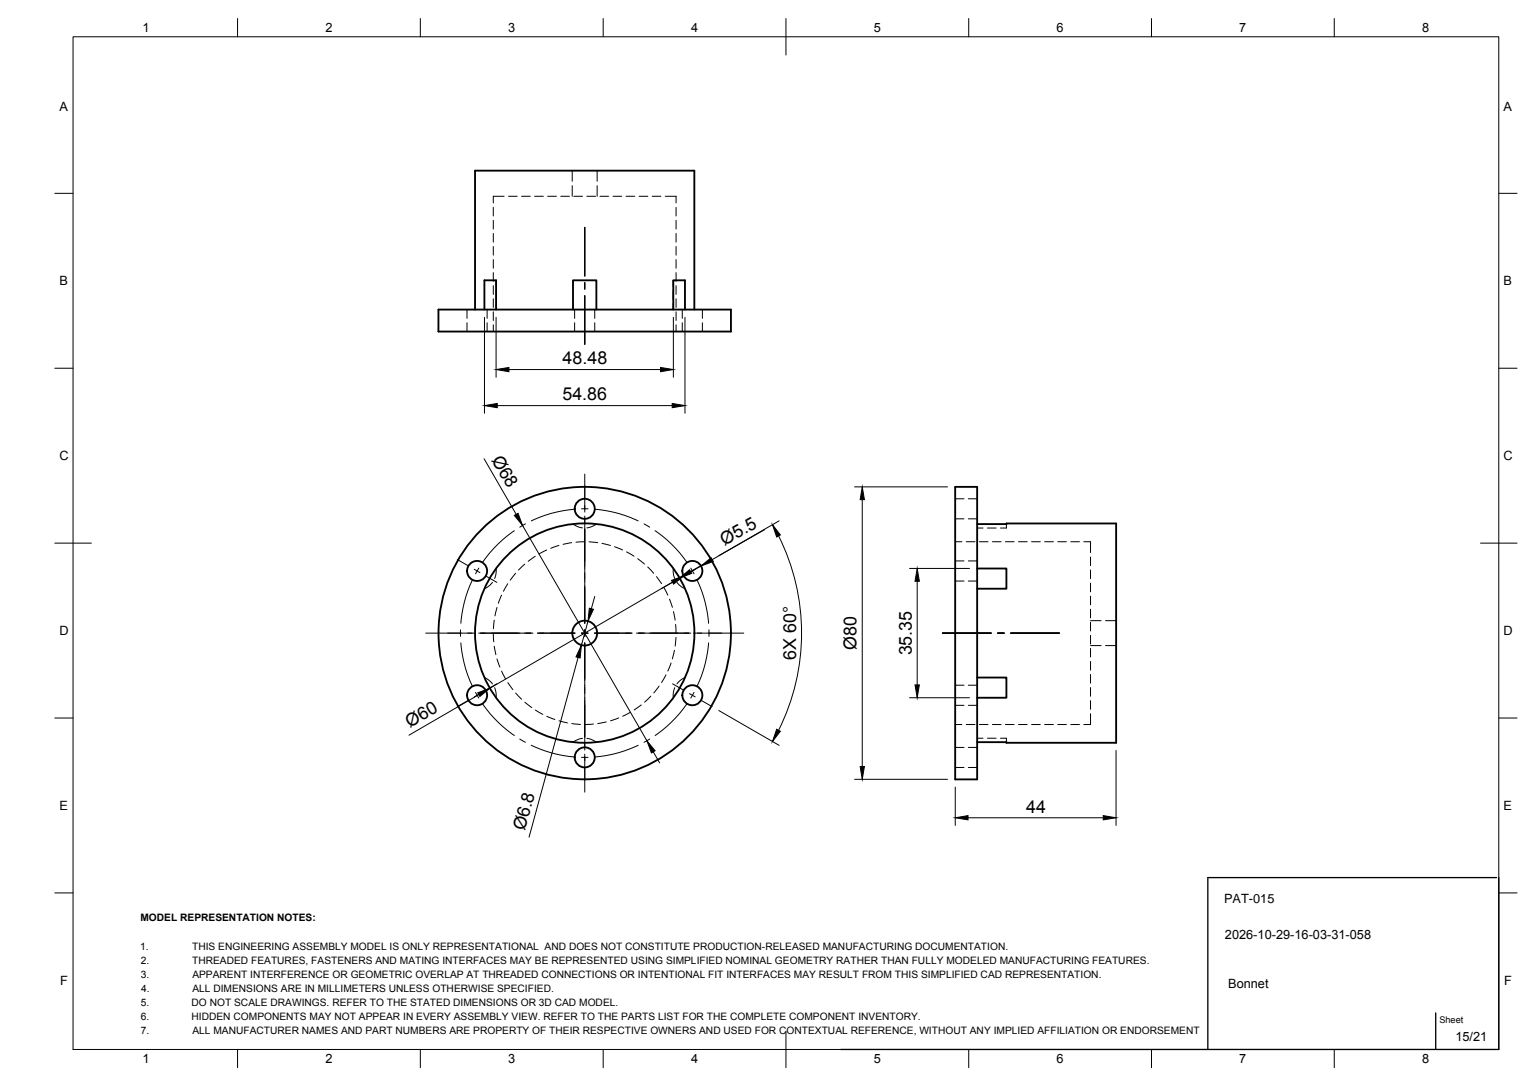
ISO-10303-21;
HEADER;
/* Generated by software containing ST-Developer
 * from STEP Tools, Inc. (www.steptools.com) 
 */

FILE_DESCRIPTION(
/* description */ ('PAT-015'),
/* implementation_level */ '2;1');

FILE_NAME(
/* name */ 'Bonnet.step',
/* time_stamp */ '2026-10-29T16:03:43-07:00',
/* author */ (''),
/* organization */ (''),
/* preprocessor_version */ 'ST-DEVELOPER v20.2',
/* originating_system */ 'Autodesk Translation Framework v15.17.0.0',
/* authorisation */ '');

FILE_SCHEMA (('AUTOMOTIVE_DESIGN { 1 0 10303 214 3 1 1 }'));
ENDSEC;

DATA;
#10=MECHANICAL_DESIGN_GEOMETRIC_PRESENTATION_REPRESENTATION('',(#243),#10266);
#195=SHAPE_REPRESENTATION_RELATIONSHIP('SRR','None',#10366,#218);
#218=ADVANCED_BREP_SHAPE_REPRESENTATION('',(#268),#10254);
#243=STYLED_ITEM('',(#10540),#268);
#268=MANIFOLD_SOLID_BREP('Body1',#4702);
#390=FACE_BOUND('',#1144,.T.);
#391=FACE_BOUND('',#1146,.T.);
#392=FACE_BOUND('',#1149,.T.);
#393=FACE_BOUND('',#1150,.T.);
#394=FACE_BOUND('',#1151,.T.);
#395=FACE_BOUND('',#1152,.T.);
#396=FACE_BOUND('',#1153,.T.);
#397=FACE_BOUND('',#1154,.T.);
#398=FACE_BOUND('',#1155,.T.);
#399=FACE_BOUND('',#1157,.T.);
#400=FACE_BOUND('',#1158,.T.);
#401=FACE_BOUND('',#1159,.T.);
#402=FACE_BOUND('',#1160,.T.);
#403=FACE_BOUND('',#1161,.T.);
#404=FACE_BOUND('',#1162,.T.);
#405=FACE_BOUND('',#1163,.T.);
#503=PLANE('',#5307);
#504=PLANE('',#5315);
#505=PLANE('',#5317);
#506=PLANE('',#5322);
#507=PLANE('',#5327);
#508=PLANE('',#5335);
#509=PLANE('',#5370);
#510=PLANE('',#5371);
#511=PLANE('',#5375);
#512=PLANE('',#5376);
#741=FACE_OUTER_BOUND('',#1122,.T.);
#742=FACE_OUTER_BOUND('',#1123,.T.);
#743=FACE_OUTER_BOUND('',#1124,.T.);
#744=FACE_OUTER_BOUND('',#1125,.T.);
#745=FACE_OUTER_BOUND('',#1126,.T.);
#746=FACE_OUTER_BOUND('',#1127,.T.);
#747=FACE_OUTER_BOUND('',#1128,.T.);
#748=FACE_OUTER_BOUND('',#1129,.T.);
#749=FACE_OUTER_BOUND('',#1130,.T.);
#750=FACE_OUTER_BOUND('',#1131,.T.);
#751=FACE_OUTER_BOUND('',#1132,.T.);
#752=FACE_OUTER_BOUND('',#1133,.T.);
#753=FACE_OUTER_BOUND('',#1134,.T.);
#754=FACE_OUTER_BOUND('',#1135,.T.);
#755=FACE_OUTER_BOUND('',#1136,.T.);
#756=FACE_OUTER_BOUND('',#1137,.T.);
#757=FACE_OUTER_BOUND('',#1138,.T.);
#758=FACE_OUTER_BOUND('',#1139,.T.);
#759=FACE_OUTER_BOUND('',#1140,.T.);
#760=FACE_OUTER_BOUND('',#1141,.T.);
#761=FACE_OUTER_BOUND('',#1142,.T.);
#762=FACE_OUTER_BOUND('',#1143,.T.);
#763=FACE_OUTER_BOUND('',#1145,.T.);
#764=FACE_OUTER_BOUND('',#1147,.T.);
#765=FACE_OUTER_BOUND('',#1148,.T.);
#766=FACE_OUTER_BOUND('',#1156,.T.);
#1122=EDGE_LOOP('',(#3831,#3832));
#1123=EDGE_LOOP('',(#3833,#3834,#3835,#3836));
#1124=EDGE_LOOP('',(#3837,#3838,#3839,#3840));
#1125=EDGE_LOOP('',(#3841,#3842));
#1126=EDGE_LOOP('',(#3843,#3844));
#1127=EDGE_LOOP('',(#3845,#3846,#3847,#3848));
#1128=EDGE_LOOP('',(#3849,#3850));
#1129=EDGE_LOOP('',(#3851,#3852,#3853,#3854));
#1130=EDGE_LOOP('',(#3855,#3856));
#1131=EDGE_LOOP('',(#3857,#3858,#3859,#3860));
#1132=EDGE_LOOP('',(#3861,#3862,#3863,#3864));
#1133=EDGE_LOOP('',(#3865,#3866));
#1134=EDGE_LOOP('',(#3867,#3868,#3869,#3870,#3871,#3872,#3873,#3874,#3875,
#3876,#3877,#3878,#3879,#3880,#3881,#3882,#3883,#3884,#3885,#3886,#3887,
#3888,#3889,#3890,#3891,#3892,#3893,#3894));
#1135=EDGE_LOOP('',(#3895,#3896,#3897,#3898));
#1136=EDGE_LOOP('',(#3899,#3900,#3901,#3902));
#1137=EDGE_LOOP('',(#3903,#3904,#3905,#3906));
#1138=EDGE_LOOP('',(#3907,#3908,#3909,#3910));
#1139=EDGE_LOOP('',(#3911,#3912,#3913,#3914));
#1140=EDGE_LOOP('',(#3915,#3916,#3917,#3918));
#1141=EDGE_LOOP('',(#3919,#3920,#3921,#3922));
#1142=EDGE_LOOP('',(#3923,#3924,#3925,#3926));
#1143=EDGE_LOOP('',(#3927));
#1144=EDGE_LOOP('',(#3928));
#1145=EDGE_LOOP('',(#3929));
#1146=EDGE_LOOP('',(#3930));
#1147=EDGE_LOOP('',(#3931,#3932,#3933,#3934));
#1148=EDGE_LOOP('',(#3935));
#1149=EDGE_LOOP('',(#3936));
#1150=EDGE_LOOP('',(#3937));
#1151=EDGE_LOOP('',(#3938));
#1152=EDGE_LOOP('',(#3939));
#1153=EDGE_LOOP('',(#3940));
#1154=EDGE_LOOP('',(#3941));
#1155=EDGE_LOOP('',(#3942,#3943,#3944,#3945,#3946,#3947,#3948,#3949,#3950,
#3951,#3952,#3953,#3954));
#1156=EDGE_LOOP('',(#3955));
#1157=EDGE_LOOP('',(#3956));
#1158=EDGE_LOOP('',(#3957));
#1159=EDGE_LOOP('',(#3958));
#1160=EDGE_LOOP('',(#3959));
#1161=EDGE_LOOP('',(#3960));
#1162=EDGE_LOOP('',(#3961));
#1163=EDGE_LOOP('',(#3962));
#1480=LINE('',#8832,#1760);
#1481=LINE('',#8835,#1761);
#1482=LINE('',#8839,#1762);
#1483=LINE('',#8843,#1763);
#1484=LINE('',#8854,#1764);
#1485=LINE('',#8857,#1765);
#1486=LINE('',#8865,#1766);
#1487=LINE('',#8868,#1767);
#1488=LINE('',#8876,#1768);
#1489=LINE('',#8879,#1769);
#1490=LINE('',#8883,#1770);
#1491=LINE('',#8887,#1771);
#1492=LINE('',#8895,#1772);
#1493=LINE('',#8907,#1773);
#1494=LINE('',#8913,#1774);
#1495=LINE('',#8919,#1775);
#1496=LINE('',#8925,#1776);
#1497=LINE('',#8931,#1777);
#1498=LINE('',#8937,#1778);
#1499=LINE('',#8943,#1779);
#1500=LINE('',#8949,#1780);
#1501=LINE('',#8957,#1781);
#1760=VECTOR('',#6395,1.);
#1761=VECTOR('',#6398,1.);
#1762=VECTOR('',#6401,1.);
#1763=VECTOR('',#6404,1.);
#1764=VECTOR('',#6419,1.);
#1765=VECTOR('',#6422,1.);
#1766=VECTOR('',#6431,1.);
#1767=VECTOR('',#6434,1.);
#1768=VECTOR('',#6443,1.);
#1769=VECTOR('',#6446,1.);
#1770=VECTOR('',#6449,1.);
#1771=VECTOR('',#6452,1.);
#1772=VECTOR('',#6463,3.);
#1773=VECTOR('',#6482,0.275);
#1774=VECTOR('',#6489,0.275);
#1775=VECTOR('',#6496,0.275);
#1776=VECTOR('',#6503,0.275);
#1777=VECTOR('',#6510,0.275);
#1778=VECTOR('',#6517,0.275);
#1779=VECTOR('',#6524,0.34);
#1780=VECTOR('',#6531,2.5);
#1781=VECTOR('',#6542,4.);
#2023=CIRCLE('',#5308,3.);
#2024=CIRCLE('',#5309,0.525);
#2025=CIRCLE('',#5311,0.525);
#2026=CIRCLE('',#5313,0.525);
#2027=CIRCLE('',#5314,0.525);
#2028=CIRCLE('',#5316,3.);
#2029=CIRCLE('',#5318,3.);
#2030=CIRCLE('',#5319,0.525);
#2031=CIRCLE('',#5321,0.525);
#2032=CIRCLE('',#5323,3.);
#2033=CIRCLE('',#5324,0.525);
#2034=CIRCLE('',#5326,0.525);
#2035=CIRCLE('',#5328,3.);
#2036=CIRCLE('',#5329,0.525);
#2037=CIRCLE('',#5331,0.525);
#2038=CIRCLE('',#5333,0.525);
#2039=CIRCLE('',#5334,0.525);
#2040=CIRCLE('',#5336,3.);
#2041=CIRCLE('',#5338,3.);
#2042=CIRCLE('',#5339,3.);
#2043=CIRCLE('',#5340,3.);
#2044=CIRCLE('',#5341,3.);
#2045=CIRCLE('',#5342,3.);
#2046=CIRCLE('',#5343,3.);
#2047=CIRCLE('',#5344,3.);
#2048=CIRCLE('',#5345,3.);
#2049=CIRCLE('',#5347,0.275);
#2050=CIRCLE('',#5348,0.275);
#2051=CIRCLE('',#5350,0.275);
#2052=CIRCLE('',#5351,0.275);
#2053=CIRCLE('',#5353,0.275);
#2054=CIRCLE('',#5354,0.275);
#2055=CIRCLE('',#5356,0.275);
#2056=CIRCLE('',#5357,0.275);
#2057=CIRCLE('',#5359,0.275);
#2058=CIRCLE('',#5360,0.275);
#2059=CIRCLE('',#5362,0.275);
#2060=CIRCLE('',#5363,0.275);
#2061=CIRCLE('',#5365,0.34);
#2062=CIRCLE('',#5366,0.34);
#2063=CIRCLE('',#5368,2.5);
#2064=CIRCLE('',#5369,2.5);
#2065=CIRCLE('',#5373,4.);
#2066=CIRCLE('',#5374,4.);
#2357=VERTEX_POINT('',#8826);
#2358=VERTEX_POINT('',#8827);
#2359=VERTEX_POINT('',#8831);
#2360=VERTEX_POINT('',#8833);
#2361=VERTEX_POINT('',#8837);
#2362=VERTEX_POINT('',#8838);
#2363=VERTEX_POINT('',#8840);
#2364=VERTEX_POINT('',#8842);
#2365=VERTEX_POINT('',#8848);
#2366=VERTEX_POINT('',#8849);
#2367=VERTEX_POINT('',#8853);
#2368=VERTEX_POINT('',#8855);
#2369=VERTEX_POINT('',#8859);
#2370=VERTEX_POINT('',#8860);
#2371=VERTEX_POINT('',#8864);
#2372=VERTEX_POINT('',#8866);
#2373=VERTEX_POINT('',#8870);
#2374=VERTEX_POINT('',#8871);
#2375=VERTEX_POINT('',#8875);
#2376=VERTEX_POINT('',#8877);
#2377=VERTEX_POINT('',#8881);
#2378=VERTEX_POINT('',#8882);
#2379=VERTEX_POINT('',#8884);
#2380=VERTEX_POINT('',#8886);
#2381=VERTEX_POINT('',#8892);
#2382=VERTEX_POINT('',#8894);
#2383=VERTEX_POINT('',#8904);
#2384=VERTEX_POINT('',#8906);
#2385=VERTEX_POINT('',#8910);
#2386=VERTEX_POINT('',#8912);
#2387=VERTEX_POINT('',#8916);
#2388=VERTEX_POINT('',#8918);
#2389=VERTEX_POINT('',#8922);
#2390=VERTEX_POINT('',#8924);
#2391=VERTEX_POINT('',#8928);
#2392=VERTEX_POINT('',#8930);
#2393=VERTEX_POINT('',#8934);
#2394=VERTEX_POINT('',#8936);
#2395=VERTEX_POINT('',#8940);
#2396=VERTEX_POINT('',#8942);
#2397=VERTEX_POINT('',#8946);
#2398=VERTEX_POINT('',#8948);
#2399=VERTEX_POINT('',#8954);
#2400=VERTEX_POINT('',#8956);
#2871=EDGE_CURVE('',#2357,#2358,#2023,.T.);
#2872=EDGE_CURVE('',#2358,#2357,#2024,.T.);
#2873=EDGE_CURVE('',#2359,#2357,#1480,.T.);
#2874=EDGE_CURVE('',#2360,#2359,#2025,.T.);
#2875=EDGE_CURVE('',#2358,#2360,#1481,.T.);
#2876=EDGE_CURVE('',#2361,#2362,#1482,.T.);
#2877=EDGE_CURVE('',#2361,#2363,#2026,.T.);
#2878=EDGE_CURVE('',#2364,#2363,#1483,.T.);
#2879=EDGE_CURVE('',#2362,#2364,#2027,.T.);
#2880=EDGE_CURVE('',#2363,#2361,#2028,.T.);
#2881=EDGE_CURVE('',#2365,#2366,#2029,.T.);
#2882=EDGE_CURVE('',#2366,#2365,#2030,.T.);
#2883=EDGE_CURVE('',#2367,#2365,#1484,.T.);
#2884=EDGE_CURVE('',#2368,#2367,#2031,.T.);
#2885=EDGE_CURVE('',#2366,#2368,#1485,.T.);
#2886=EDGE_CURVE('',#2369,#2370,#2032,.T.);
#2887=EDGE_CURVE('',#2370,#2369,#2033,.T.);
#2888=EDGE_CURVE('',#2371,#2369,#1486,.T.);
#2889=EDGE_CURVE('',#2372,#2371,#2034,.T.);
#2890=EDGE_CURVE('',#2370,#2372,#1487,.T.);
#2891=EDGE_CURVE('',#2373,#2374,#2035,.T.);
#2892=EDGE_CURVE('',#2374,#2373,#2036,.T.);
#2893=EDGE_CURVE('',#2375,#2373,#1488,.T.);
#2894=EDGE_CURVE('',#2376,#2375,#2037,.T.);
#2895=EDGE_CURVE('',#2374,#2376,#1489,.T.);
#2896=EDGE_CURVE('',#2377,#2378,#1490,.T.);
#2897=EDGE_CURVE('',#2377,#2379,#2038,.T.);
#2898=EDGE_CURVE('',#2380,#2379,#1491,.T.);
#2899=EDGE_CURVE('',#2378,#2380,#2039,.T.);
#2900=EDGE_CURVE('',#2379,#2377,#2040,.T.);
#2901=EDGE_CURVE('',#2381,#2381,#2041,.T.);
#2902=EDGE_CURVE('',#2381,#2382,#1492,.T.);
#2903=EDGE_CURVE('',#2375,#2382,#2042,.T.);
#2904=EDGE_CURVE('',#2359,#2376,#2043,.T.);
#2905=EDGE_CURVE('',#2380,#2360,#2044,.T.);
#2906=EDGE_CURVE('',#2364,#2378,#2045,.T.);
#2907=EDGE_CURVE('',#2367,#2362,#2046,.T.);
#2908=EDGE_CURVE('',#2371,#2368,#2047,.T.);
#2909=EDGE_CURVE('',#2382,#2372,#2048,.T.);
#2910=EDGE_CURVE('',#2383,#2383,#2049,.T.);
#2911=EDGE_CURVE('',#2383,#2384,#1493,.T.);
#2912=EDGE_CURVE('',#2384,#2384,#2050,.T.);
#2913=EDGE_CURVE('',#2385,#2385,#2051,.T.);
#2914=EDGE_CURVE('',#2385,#2386,#1494,.T.);
#2915=EDGE_CURVE('',#2386,#2386,#2052,.T.);
#2916=EDGE_CURVE('',#2387,#2387,#2053,.T.);
#2917=EDGE_CURVE('',#2387,#2388,#1495,.T.);
#2918=EDGE_CURVE('',#2388,#2388,#2054,.T.);
#2919=EDGE_CURVE('',#2389,#2389,#2055,.T.);
#2920=EDGE_CURVE('',#2389,#2390,#1496,.T.);
#2921=EDGE_CURVE('',#2390,#2390,#2056,.T.);
#2922=EDGE_CURVE('',#2391,#2391,#2057,.T.);
#2923=EDGE_CURVE('',#2391,#2392,#1497,.T.);
#2924=EDGE_CURVE('',#2392,#2392,#2058,.T.);
#2925=EDGE_CURVE('',#2393,#2393,#2059,.T.);
#2926=EDGE_CURVE('',#2393,#2394,#1498,.T.);
#2927=EDGE_CURVE('',#2394,#2394,#2060,.T.);
#2928=EDGE_CURVE('',#2395,#2395,#2061,.T.);
#2929=EDGE_CURVE('',#2395,#2396,#1499,.T.);
#2930=EDGE_CURVE('',#2396,#2396,#2062,.T.);
#2931=EDGE_CURVE('',#2397,#2397,#2063,.T.);
#2932=EDGE_CURVE('',#2397,#2398,#1500,.T.);
#2933=EDGE_CURVE('',#2398,#2398,#2064,.T.);
#2934=EDGE_CURVE('',#2399,#2399,#2065,.T.);
#2935=EDGE_CURVE('',#2399,#2400,#1501,.T.);
#2936=EDGE_CURVE('',#2400,#2400,#2066,.T.);
#3831=ORIENTED_EDGE('',*,*,#2871,.F.);
#3832=ORIENTED_EDGE('',*,*,#2872,.F.);
#3833=ORIENTED_EDGE('',*,*,#2873,.F.);
#3834=ORIENTED_EDGE('',*,*,#2874,.F.);
#3835=ORIENTED_EDGE('',*,*,#2875,.F.);
#3836=ORIENTED_EDGE('',*,*,#2872,.T.);
#3837=ORIENTED_EDGE('',*,*,#2876,.F.);
#3838=ORIENTED_EDGE('',*,*,#2877,.T.);
#3839=ORIENTED_EDGE('',*,*,#2878,.F.);
#3840=ORIENTED_EDGE('',*,*,#2879,.F.);
#3841=ORIENTED_EDGE('',*,*,#2880,.F.);
#3842=ORIENTED_EDGE('',*,*,#2877,.F.);
#3843=ORIENTED_EDGE('',*,*,#2881,.F.);
#3844=ORIENTED_EDGE('',*,*,#2882,.F.);
#3845=ORIENTED_EDGE('',*,*,#2883,.F.);
#3846=ORIENTED_EDGE('',*,*,#2884,.F.);
#3847=ORIENTED_EDGE('',*,*,#2885,.F.);
#3848=ORIENTED_EDGE('',*,*,#2882,.T.);
#3849=ORIENTED_EDGE('',*,*,#2886,.F.);
#3850=ORIENTED_EDGE('',*,*,#2887,.F.);
#3851=ORIENTED_EDGE('',*,*,#2888,.F.);
#3852=ORIENTED_EDGE('',*,*,#2889,.F.);
#3853=ORIENTED_EDGE('',*,*,#2890,.F.);
#3854=ORIENTED_EDGE('',*,*,#2887,.T.);
#3855=ORIENTED_EDGE('',*,*,#2891,.F.);
#3856=ORIENTED_EDGE('',*,*,#2892,.F.);
#3857=ORIENTED_EDGE('',*,*,#2893,.F.);
#3858=ORIENTED_EDGE('',*,*,#2894,.F.);
#3859=ORIENTED_EDGE('',*,*,#2895,.F.);
#3860=ORIENTED_EDGE('',*,*,#2892,.T.);
#3861=ORIENTED_EDGE('',*,*,#2896,.F.);
#3862=ORIENTED_EDGE('',*,*,#2897,.T.);
#3863=ORIENTED_EDGE('',*,*,#2898,.F.);
#3864=ORIENTED_EDGE('',*,*,#2899,.F.);
#3865=ORIENTED_EDGE('',*,*,#2900,.F.);
#3866=ORIENTED_EDGE('',*,*,#2897,.F.);
#3867=ORIENTED_EDGE('',*,*,#2901,.F.);
#3868=ORIENTED_EDGE('',*,*,#2902,.T.);
#3869=ORIENTED_EDGE('',*,*,#2903,.F.);
#3870=ORIENTED_EDGE('',*,*,#2893,.T.);
#3871=ORIENTED_EDGE('',*,*,#2891,.T.);
#3872=ORIENTED_EDGE('',*,*,#2895,.T.);
#3873=ORIENTED_EDGE('',*,*,#2904,.F.);
#3874=ORIENTED_EDGE('',*,*,#2873,.T.);
#3875=ORIENTED_EDGE('',*,*,#2871,.T.);
#3876=ORIENTED_EDGE('',*,*,#2875,.T.);
#3877=ORIENTED_EDGE('',*,*,#2905,.F.);
#3878=ORIENTED_EDGE('',*,*,#2898,.T.);
#3879=ORIENTED_EDGE('',*,*,#2900,.T.);
#3880=ORIENTED_EDGE('',*,*,#2896,.T.);
#3881=ORIENTED_EDGE('',*,*,#2906,.F.);
#3882=ORIENTED_EDGE('',*,*,#2878,.T.);
#3883=ORIENTED_EDGE('',*,*,#2880,.T.);
#3884=ORIENTED_EDGE('',*,*,#2876,.T.);
#3885=ORIENTED_EDGE('',*,*,#2907,.F.);
#3886=ORIENTED_EDGE('',*,*,#2883,.T.);
#3887=ORIENTED_EDGE('',*,*,#2881,.T.);
#3888=ORIENTED_EDGE('',*,*,#2885,.T.);
#3889=ORIENTED_EDGE('',*,*,#2908,.F.);
#3890=ORIENTED_EDGE('',*,*,#2888,.T.);
#3891=ORIENTED_EDGE('',*,*,#2886,.T.);
#3892=ORIENTED_EDGE('',*,*,#2890,.T.);
#3893=ORIENTED_EDGE('',*,*,#2909,.F.);
#3894=ORIENTED_EDGE('',*,*,#2902,.F.);
#3895=ORIENTED_EDGE('',*,*,#2910,.F.);
#3896=ORIENTED_EDGE('',*,*,#2911,.T.);
#3897=ORIENTED_EDGE('',*,*,#2912,.F.);
#3898=ORIENTED_EDGE('',*,*,#2911,.F.);
#3899=ORIENTED_EDGE('',*,*,#2913,.F.);
#3900=ORIENTED_EDGE('',*,*,#2914,.T.);
#3901=ORIENTED_EDGE('',*,*,#2915,.F.);
#3902=ORIENTED_EDGE('',*,*,#2914,.F.);
#3903=ORIENTED_EDGE('',*,*,#2916,.F.);
#3904=ORIENTED_EDGE('',*,*,#2917,.T.);
#3905=ORIENTED_EDGE('',*,*,#2918,.F.);
#3906=ORIENTED_EDGE('',*,*,#2917,.F.);
#3907=ORIENTED_EDGE('',*,*,#2919,.F.);
#3908=ORIENTED_EDGE('',*,*,#2920,.T.);
#3909=ORIENTED_EDGE('',*,*,#2921,.F.);
#3910=ORIENTED_EDGE('',*,*,#2920,.F.);
#3911=ORIENTED_EDGE('',*,*,#2922,.F.);
#3912=ORIENTED_EDGE('',*,*,#2923,.T.);
#3913=ORIENTED_EDGE('',*,*,#2924,.F.);
#3914=ORIENTED_EDGE('',*,*,#2923,.F.);
#3915=ORIENTED_EDGE('',*,*,#2925,.F.);
#3916=ORIENTED_EDGE('',*,*,#2926,.T.);
#3917=ORIENTED_EDGE('',*,*,#2927,.F.);
#3918=ORIENTED_EDGE('',*,*,#2926,.F.);
#3919=ORIENTED_EDGE('',*,*,#2928,.F.);
#3920=ORIENTED_EDGE('',*,*,#2929,.T.);
#3921=ORIENTED_EDGE('',*,*,#2930,.F.);
#3922=ORIENTED_EDGE('',*,*,#2929,.F.);
#3923=ORIENTED_EDGE('',*,*,#2931,.F.);
#3924=ORIENTED_EDGE('',*,*,#2932,.T.);
#3925=ORIENTED_EDGE('',*,*,#2933,.T.);
#3926=ORIENTED_EDGE('',*,*,#2932,.F.);
#3927=ORIENTED_EDGE('',*,*,#2933,.F.);
#3928=ORIENTED_EDGE('',*,*,#2928,.T.);
#3929=ORIENTED_EDGE('',*,*,#2901,.T.);
#3930=ORIENTED_EDGE('',*,*,#2930,.T.);
#3931=ORIENTED_EDGE('',*,*,#2934,.F.);
#3932=ORIENTED_EDGE('',*,*,#2935,.T.);
#3933=ORIENTED_EDGE('',*,*,#2936,.T.);
#3934=ORIENTED_EDGE('',*,*,#2935,.F.);
#3935=ORIENTED_EDGE('',*,*,#2934,.T.);
#3936=ORIENTED_EDGE('',*,*,#2912,.T.);
#3937=ORIENTED_EDGE('',*,*,#2915,.T.);
#3938=ORIENTED_EDGE('',*,*,#2918,.T.);
#3939=ORIENTED_EDGE('',*,*,#2921,.T.);
#3940=ORIENTED_EDGE('',*,*,#2924,.T.);
#3941=ORIENTED_EDGE('',*,*,#2927,.T.);
#3942=ORIENTED_EDGE('',*,*,#2904,.T.);
#3943=ORIENTED_EDGE('',*,*,#2894,.T.);
#3944=ORIENTED_EDGE('',*,*,#2903,.T.);
#3945=ORIENTED_EDGE('',*,*,#2909,.T.);
#3946=ORIENTED_EDGE('',*,*,#2889,.T.);
#3947=ORIENTED_EDGE('',*,*,#2908,.T.);
#3948=ORIENTED_EDGE('',*,*,#2884,.T.);
#3949=ORIENTED_EDGE('',*,*,#2907,.T.);
#3950=ORIENTED_EDGE('',*,*,#2879,.T.);
#3951=ORIENTED_EDGE('',*,*,#2906,.T.);
#3952=ORIENTED_EDGE('',*,*,#2899,.T.);
#3953=ORIENTED_EDGE('',*,*,#2905,.T.);
#3954=ORIENTED_EDGE('',*,*,#2874,.T.);
#3955=ORIENTED_EDGE('',*,*,#2936,.F.);
#3956=ORIENTED_EDGE('',*,*,#2931,.T.);
#3957=ORIENTED_EDGE('',*,*,#2925,.T.);
#3958=ORIENTED_EDGE('',*,*,#2922,.T.);
#3959=ORIENTED_EDGE('',*,*,#2919,.T.);
#3960=ORIENTED_EDGE('',*,*,#2916,.T.);
#3961=ORIENTED_EDGE('',*,*,#2913,.T.);
#3962=ORIENTED_EDGE('',*,*,#2910,.T.);
#4375=CYLINDRICAL_SURFACE('',#5310,0.525);
#4376=CYLINDRICAL_SURFACE('',#5312,0.525);
#4377=CYLINDRICAL_SURFACE('',#5320,0.525);
#4378=CYLINDRICAL_SURFACE('',#5325,0.525);
#4379=CYLINDRICAL_SURFACE('',#5330,0.525);
#4380=CYLINDRICAL_SURFACE('',#5332,0.525);
#4381=CYLINDRICAL_SURFACE('',#5337,3.);
#4382=CYLINDRICAL_SURFACE('',#5346,0.275);
#4383=CYLINDRICAL_SURFACE('',#5349,0.275);
#4384=CYLINDRICAL_SURFACE('',#5352,0.275);
#4385=CYLINDRICAL_SURFACE('',#5355,0.275);
#4386=CYLINDRICAL_SURFACE('',#5358,0.275);
#4387=CYLINDRICAL_SURFACE('',#5361,0.275);
#4388=CYLINDRICAL_SURFACE('',#5364,0.34);
#4389=CYLINDRICAL_SURFACE('',#5367,2.5);
#4390=CYLINDRICAL_SURFACE('',#5372,4.);
#4576=ADVANCED_FACE('',(#741),#503,.F.);
#4577=ADVANCED_FACE('',(#742),#4375,.F.);
#4578=ADVANCED_FACE('',(#743),#4376,.F.);
#4579=ADVANCED_FACE('',(#744),#504,.F.);
#4580=ADVANCED_FACE('',(#745),#505,.F.);
#4581=ADVANCED_FACE('',(#746),#4377,.F.);
#4582=ADVANCED_FACE('',(#747),#506,.F.);
#4583=ADVANCED_FACE('',(#748),#4378,.F.);
#4584=ADVANCED_FACE('',(#749),#507,.F.);
#4585=ADVANCED_FACE('',(#750),#4379,.F.);
#4586=ADVANCED_FACE('',(#751),#4380,.F.);
#4587=ADVANCED_FACE('',(#752),#508,.F.);
#4588=ADVANCED_FACE('',(#753),#4381,.T.);
#4589=ADVANCED_FACE('',(#754),#4382,.F.);
#4590=ADVANCED_FACE('',(#755),#4383,.F.);
#4591=ADVANCED_FACE('',(#756),#4384,.F.);
#4592=ADVANCED_FACE('',(#757),#4385,.F.);
#4593=ADVANCED_FACE('',(#758),#4386,.F.);
#4594=ADVANCED_FACE('',(#759),#4387,.F.);
#4595=ADVANCED_FACE('',(#760),#4388,.F.);
#4596=ADVANCED_FACE('',(#761),#4389,.F.);
#4597=ADVANCED_FACE('',(#762,#390),#509,.F.);
#4598=ADVANCED_FACE('',(#763,#391),#510,.T.);
#4599=ADVANCED_FACE('',(#764),#4390,.T.);
#4600=ADVANCED_FACE('',(#765,#392,#393,#394,#395,#396,#397,#398),#511,.T.);
#4601=ADVANCED_FACE('',(#766,#399,#400,#401,#402,#403,#404,#405),#512,.F.);
#4702=CLOSED_SHELL('',(#4576,#4577,#4578,#4579,#4580,#4581,#4582,#4583,
#4584,#4585,#4586,#4587,#4588,#4589,#4590,#4591,#4592,#4593,#4594,#4595,
#4596,#4597,#4598,#4599,#4600,#4601));
#5306=AXIS2_PLACEMENT_3D('',#8824,#6385,#6386);
#5307=AXIS2_PLACEMENT_3D('',#8825,#6387,#6388);
#5308=AXIS2_PLACEMENT_3D('',#8828,#6389,#6390);
#5309=AXIS2_PLACEMENT_3D('',#8829,#6391,#6392);
#5310=AXIS2_PLACEMENT_3D('',#8830,#6393,#6394);
#5311=AXIS2_PLACEMENT_3D('',#8834,#6396,#6397);
#5312=AXIS2_PLACEMENT_3D('',#8836,#6399,#6400);
#5313=AXIS2_PLACEMENT_3D('',#8841,#6402,#6403);
#5314=AXIS2_PLACEMENT_3D('',#8844,#6405,#6406);
#5315=AXIS2_PLACEMENT_3D('',#8845,#6407,#6408);
#5316=AXIS2_PLACEMENT_3D('',#8846,#6409,#6410);
#5317=AXIS2_PLACEMENT_3D('',#8847,#6411,#6412);
#5318=AXIS2_PLACEMENT_3D('',#8850,#6413,#6414);
#5319=AXIS2_PLACEMENT_3D('',#8851,#6415,#6416);
#5320=AXIS2_PLACEMENT_3D('',#8852,#6417,#6418);
#5321=AXIS2_PLACEMENT_3D('',#8856,#6420,#6421);
#5322=AXIS2_PLACEMENT_3D('',#8858,#6423,#6424);
#5323=AXIS2_PLACEMENT_3D('',#8861,#6425,#6426);
#5324=AXIS2_PLACEMENT_3D('',#8862,#6427,#6428);
#5325=AXIS2_PLACEMENT_3D('',#8863,#6429,#6430);
#5326=AXIS2_PLACEMENT_3D('',#8867,#6432,#6433);
#5327=AXIS2_PLACEMENT_3D('',#8869,#6435,#6436);
#5328=AXIS2_PLACEMENT_3D('',#8872,#6437,#6438);
#5329=AXIS2_PLACEMENT_3D('',#8873,#6439,#6440);
#5330=AXIS2_PLACEMENT_3D('',#8874,#6441,#6442);
#5331=AXIS2_PLACEMENT_3D('',#8878,#6444,#6445);
#5332=AXIS2_PLACEMENT_3D('',#8880,#6447,#6448);
#5333=AXIS2_PLACEMENT_3D('',#8885,#6450,#6451);
#5334=AXIS2_PLACEMENT_3D('',#8888,#6453,#6454);
#5335=AXIS2_PLACEMENT_3D('',#8889,#6455,#6456);
#5336=AXIS2_PLACEMENT_3D('',#8890,#6457,#6458);
#5337=AXIS2_PLACEMENT_3D('',#8891,#6459,#6460);
#5338=AXIS2_PLACEMENT_3D('',#8893,#6461,#6462);
#5339=AXIS2_PLACEMENT_3D('',#8896,#6464,#6465);
#5340=AXIS2_PLACEMENT_3D('',#8897,#6466,#6467);
#5341=AXIS2_PLACEMENT_3D('',#8898,#6468,#6469);
#5342=AXIS2_PLACEMENT_3D('',#8899,#6470,#6471);
#5343=AXIS2_PLACEMENT_3D('',#8900,#6472,#6473);
#5344=AXIS2_PLACEMENT_3D('',#8901,#6474,#6475);
#5345=AXIS2_PLACEMENT_3D('',#8902,#6476,#6477);
#5346=AXIS2_PLACEMENT_3D('',#8903,#6478,#6479);
#5347=AXIS2_PLACEMENT_3D('',#8905,#6480,#6481);
#5348=AXIS2_PLACEMENT_3D('',#8908,#6483,#6484);
#5349=AXIS2_PLACEMENT_3D('',#8909,#6485,#6486);
#5350=AXIS2_PLACEMENT_3D('',#8911,#6487,#6488);
#5351=AXIS2_PLACEMENT_3D('',#8914,#6490,#6491);
#5352=AXIS2_PLACEMENT_3D('',#8915,#6492,#6493);
#5353=AXIS2_PLACEMENT_3D('',#8917,#6494,#6495);
#5354=AXIS2_PLACEMENT_3D('',#8920,#6497,#6498);
#5355=AXIS2_PLACEMENT_3D('',#8921,#6499,#6500);
#5356=AXIS2_PLACEMENT_3D('',#8923,#6501,#6502);
#5357=AXIS2_PLACEMENT_3D('',#8926,#6504,#6505);
#5358=AXIS2_PLACEMENT_3D('',#8927,#6506,#6507);
#5359=AXIS2_PLACEMENT_3D('',#8929,#6508,#6509);
#5360=AXIS2_PLACEMENT_3D('',#8932,#6511,#6512);
#5361=AXIS2_PLACEMENT_3D('',#8933,#6513,#6514);
#5362=AXIS2_PLACEMENT_3D('',#8935,#6515,#6516);
#5363=AXIS2_PLACEMENT_3D('',#8938,#6518,#6519);
#5364=AXIS2_PLACEMENT_3D('',#8939,#6520,#6521);
#5365=AXIS2_PLACEMENT_3D('',#8941,#6522,#6523);
#5366=AXIS2_PLACEMENT_3D('',#8944,#6525,#6526);
#5367=AXIS2_PLACEMENT_3D('',#8945,#6527,#6528);
#5368=AXIS2_PLACEMENT_3D('',#8947,#6529,#6530);
#5369=AXIS2_PLACEMENT_3D('',#8950,#6532,#6533);
#5370=AXIS2_PLACEMENT_3D('',#8951,#6534,#6535);
#5371=AXIS2_PLACEMENT_3D('',#8952,#6536,#6537);
#5372=AXIS2_PLACEMENT_3D('',#8953,#6538,#6539);
#5373=AXIS2_PLACEMENT_3D('',#8955,#6540,#6541);
#5374=AXIS2_PLACEMENT_3D('',#8958,#6543,#6544);
#5375=AXIS2_PLACEMENT_3D('',#8959,#6545,#6546);
#5376=AXIS2_PLACEMENT_3D('',#8960,#6547,#6548);
#6385=DIRECTION('axis',(0.,0.,1.));
#6386=DIRECTION('refdir',(1.,0.,0.));
#6387=DIRECTION('center_axis',(0.,0.,1.));
#6388=DIRECTION('ref_axis',(1.,0.,0.));
#6389=DIRECTION('center_axis',(0.,0.,1.));
#6390=DIRECTION('ref_axis',(1.,0.,0.));
#6391=DIRECTION('center_axis',(0.,0.,1.));
#6392=DIRECTION('ref_axis',(1.,0.,0.));
#6393=DIRECTION('center_axis',(0.,0.,1.));
#6394=DIRECTION('ref_axis',(1.,0.,0.));
#6395=DIRECTION('',(0.,0.,1.));
#6396=DIRECTION('center_axis',(0.,0.,1.));
#6397=DIRECTION('ref_axis',(1.,0.,0.));
#6398=DIRECTION('',(0.,0.,-1.));
#6399=DIRECTION('center_axis',(0.,0.,1.));
#6400=DIRECTION('ref_axis',(-0.866025403784439,-0.5,0.));
#6401=DIRECTION('',(0.,0.,-1.));
#6402=DIRECTION('center_axis',(0.,0.,1.));
#6403=DIRECTION('ref_axis',(1.,0.,0.));
#6404=DIRECTION('',(0.,0.,1.));
#6405=DIRECTION('center_axis',(0.,0.,1.));
#6406=DIRECTION('ref_axis',(1.,0.,0.));
#6407=DIRECTION('center_axis',(0.,0.,1.));
#6408=DIRECTION('ref_axis',(1.,0.,0.));
#6409=DIRECTION('center_axis',(0.,0.,1.));
#6410=DIRECTION('ref_axis',(1.,0.,0.));
#6411=DIRECTION('center_axis',(0.,0.,1.));
#6412=DIRECTION('ref_axis',(1.,0.,0.));
#6413=DIRECTION('center_axis',(0.,0.,1.));
#6414=DIRECTION('ref_axis',(1.,0.,0.));
#6415=DIRECTION('center_axis',(0.,0.,1.));
#6416=DIRECTION('ref_axis',(1.,0.,0.));
#6417=DIRECTION('center_axis',(0.,0.,1.));
#6418=DIRECTION('ref_axis',(1.,0.,0.));
#6419=DIRECTION('',(0.,0.,1.));
#6420=DIRECTION('center_axis',(0.,0.,1.));
#6421=DIRECTION('ref_axis',(1.,0.,0.));
#6422=DIRECTION('',(0.,0.,-1.));
#6423=DIRECTION('center_axis',(0.,0.,1.));
#6424=DIRECTION('ref_axis',(1.,0.,0.));
#6425=DIRECTION('center_axis',(0.,0.,1.));
#6426=DIRECTION('ref_axis',(1.,0.,0.));
#6427=DIRECTION('center_axis',(0.,0.,1.));
#6428=DIRECTION('ref_axis',(1.,0.,0.));
#6429=DIRECTION('center_axis',(0.,0.,1.));
#6430=DIRECTION('ref_axis',(1.,0.,0.));
#6431=DIRECTION('',(0.,0.,1.));
#6432=DIRECTION('center_axis',(0.,0.,1.));
#6433=DIRECTION('ref_axis',(1.,0.,0.));
#6434=DIRECTION('',(0.,0.,-1.));
#6435=DIRECTION('center_axis',(0.,0.,1.));
#6436=DIRECTION('ref_axis',(1.,0.,0.));
#6437=DIRECTION('center_axis',(0.,0.,1.));
#6438=DIRECTION('ref_axis',(1.,0.,0.));
#6439=DIRECTION('center_axis',(0.,0.,1.));
#6440=DIRECTION('ref_axis',(1.,0.,0.));
#6441=DIRECTION('center_axis',(0.,0.,1.));
#6442=DIRECTION('ref_axis',(1.,0.,0.));
#6443=DIRECTION('',(0.,0.,1.));
#6444=DIRECTION('center_axis',(0.,0.,1.));
#6445=DIRECTION('ref_axis',(1.,0.,0.));
#6446=DIRECTION('',(0.,0.,-1.));
#6447=DIRECTION('center_axis',(0.,0.,1.));
#6448=DIRECTION('ref_axis',(-0.866025403784438,0.5,0.));
#6449=DIRECTION('',(0.,0.,-1.));
#6450=DIRECTION('center_axis',(0.,0.,1.));
#6451=DIRECTION('ref_axis',(1.,0.,0.));
#6452=DIRECTION('',(0.,0.,1.));
#6453=DIRECTION('center_axis',(0.,0.,1.));
#6454=DIRECTION('ref_axis',(1.,0.,0.));
#6455=DIRECTION('center_axis',(0.,0.,1.));
#6456=DIRECTION('ref_axis',(1.,0.,0.));
#6457=DIRECTION('center_axis',(0.,0.,1.));
#6458=DIRECTION('ref_axis',(1.,0.,0.));
#6459=DIRECTION('center_axis',(0.,0.,1.));
#6460=DIRECTION('ref_axis',(1.,0.,0.));
#6461=DIRECTION('center_axis',(0.,0.,1.));
#6462=DIRECTION('ref_axis',(1.,0.,0.));
#6463=DIRECTION('',(0.,0.,-1.));
#6464=DIRECTION('center_axis',(0.,0.,-1.));
#6465=DIRECTION('ref_axis',(1.,0.,0.));
#6466=DIRECTION('center_axis',(0.,0.,-1.));
#6467=DIRECTION('ref_axis',(1.,0.,0.));
#6468=DIRECTION('center_axis',(0.,0.,-1.));
#6469=DIRECTION('ref_axis',(1.,0.,0.));
#6470=DIRECTION('center_axis',(0.,0.,-1.));
#6471=DIRECTION('ref_axis',(1.,0.,0.));
#6472=DIRECTION('center_axis',(0.,0.,-1.));
#6473=DIRECTION('ref_axis',(1.,0.,0.));
#6474=DIRECTION('center_axis',(0.,0.,-1.));
#6475=DIRECTION('ref_axis',(1.,0.,0.));
#6476=DIRECTION('center_axis',(0.,0.,-1.));
#6477=DIRECTION('ref_axis',(1.,0.,0.));
#6478=DIRECTION('center_axis',(0.,0.,1.));
#6479=DIRECTION('ref_axis',(1.,0.,0.));
#6480=DIRECTION('center_axis',(0.,0.,1.));
#6481=DIRECTION('ref_axis',(1.,0.,0.));
#6482=DIRECTION('',(0.,0.,1.));
#6483=DIRECTION('center_axis',(0.,0.,-1.));
#6484=DIRECTION('ref_axis',(1.,0.,0.));
#6485=DIRECTION('center_axis',(0.,0.,1.));
#6486=DIRECTION('ref_axis',(1.,0.,0.));
#6487=DIRECTION('center_axis',(0.,0.,1.));
#6488=DIRECTION('ref_axis',(1.,0.,0.));
#6489=DIRECTION('',(0.,0.,1.));
#6490=DIRECTION('center_axis',(0.,0.,-1.));
#6491=DIRECTION('ref_axis',(1.,0.,0.));
#6492=DIRECTION('center_axis',(0.,0.,1.));
#6493=DIRECTION('ref_axis',(1.,0.,0.));
#6494=DIRECTION('center_axis',(0.,0.,1.));
#6495=DIRECTION('ref_axis',(1.,0.,0.));
#6496=DIRECTION('',(0.,0.,1.));
#6497=DIRECTION('center_axis',(0.,0.,-1.));
#6498=DIRECTION('ref_axis',(1.,0.,0.));
#6499=DIRECTION('center_axis',(0.,0.,1.));
#6500=DIRECTION('ref_axis',(1.,0.,0.));
#6501=DIRECTION('center_axis',(0.,0.,1.));
#6502=DIRECTION('ref_axis',(1.,0.,0.));
#6503=DIRECTION('',(0.,0.,1.));
#6504=DIRECTION('center_axis',(0.,0.,-1.));
#6505=DIRECTION('ref_axis',(1.,0.,0.));
#6506=DIRECTION('center_axis',(0.,0.,1.));
#6507=DIRECTION('ref_axis',(1.,0.,0.));
#6508=DIRECTION('center_axis',(0.,0.,1.));
#6509=DIRECTION('ref_axis',(1.,0.,0.));
#6510=DIRECTION('',(0.,0.,1.));
#6511=DIRECTION('center_axis',(0.,0.,-1.));
#6512=DIRECTION('ref_axis',(1.,0.,0.));
#6513=DIRECTION('center_axis',(0.,0.,1.));
#6514=DIRECTION('ref_axis',(1.,0.,0.));
#6515=DIRECTION('center_axis',(0.,0.,1.));
#6516=DIRECTION('ref_axis',(1.,0.,0.));
#6517=DIRECTION('',(0.,0.,1.));
#6518=DIRECTION('center_axis',(0.,0.,-1.));
#6519=DIRECTION('ref_axis',(1.,0.,0.));
#6520=DIRECTION('center_axis',(0.,0.,1.));
#6521=DIRECTION('ref_axis',(1.,0.,0.));
#6522=DIRECTION('center_axis',(0.,0.,1.));
#6523=DIRECTION('ref_axis',(1.,0.,0.));
#6524=DIRECTION('',(0.,0.,1.));
#6525=DIRECTION('center_axis',(0.,0.,-1.));
#6526=DIRECTION('ref_axis',(1.,0.,0.));
#6527=DIRECTION('center_axis',(0.,0.,1.));
#6528=DIRECTION('ref_axis',(1.,0.,0.));
#6529=DIRECTION('center_axis',(0.,0.,1.));
#6530=DIRECTION('ref_axis',(1.,0.,0.));
#6531=DIRECTION('',(0.,0.,1.));
#6532=DIRECTION('center_axis',(0.,0.,1.));
#6533=DIRECTION('ref_axis',(1.,0.,0.));
#6534=DIRECTION('center_axis',(0.,0.,1.));
#6535=DIRECTION('ref_axis',(1.,0.,0.));
#6536=DIRECTION('center_axis',(0.,0.,1.));
#6537=DIRECTION('ref_axis',(1.,0.,0.));
#6538=DIRECTION('center_axis',(0.,0.,1.));
#6539=DIRECTION('ref_axis',(1.,0.,0.));
#6540=DIRECTION('center_axis',(0.,0.,1.));
#6541=DIRECTION('ref_axis',(1.,0.,0.));
#6542=DIRECTION('',(0.,0.,-1.));
#6543=DIRECTION('center_axis',(0.,0.,1.));
#6544=DIRECTION('ref_axis',(1.,0.,0.));
#6545=DIRECTION('center_axis',(0.,0.,1.));
#6546=DIRECTION('ref_axis',(1.,0.,0.));
#6547=DIRECTION('center_axis',(0.,0.,1.));
#6548=DIRECTION('ref_axis',(1.,0.,0.));
#8824=CARTESIAN_POINT('',(0.,0.,0.));
#8825=CARTESIAN_POINT('Origin',(-6.66133814775094E-16,-3.4,6.5));
#8826=CARTESIAN_POINT('',(-0.318956006072959,-2.98299632352941,6.5));
#8827=CARTESIAN_POINT('',(0.318956006072958,-2.98299632352941,6.5));
#8828=CARTESIAN_POINT('Origin',(0.,0.,6.5));
#8829=CARTESIAN_POINT('Origin',(-6.2456986756515E-16,-3.4,6.5));
#8830=CARTESIAN_POINT('Origin',(-6.2456986756515E-16,-3.4,5.7));
#8831=CARTESIAN_POINT('',(-0.318956006072959,-2.98299632352941,5.7));
#8832=CARTESIAN_POINT('',(-0.318956006072959,-2.98299632352941,5.7));
#8833=CARTESIAN_POINT('',(0.318956006072958,-2.98299632352941,5.7));
#8834=CARTESIAN_POINT('Origin',(-6.2456986756515E-16,-3.4,5.7));
#8835=CARTESIAN_POINT('',(0.318956006072958,-2.98299632352941,5.7));
#8836=CARTESIAN_POINT('Origin',(2.94448637286709,1.7,5.7));
#8837=CARTESIAN_POINT('',(2.42387259253558,1.76772216571351,6.5));
#8838=CARTESIAN_POINT('',(2.42387259253558,1.76772216571351,5.7));
#8839=CARTESIAN_POINT('',(2.42387259253558,1.76772216571351,5.7));
#8840=CARTESIAN_POINT('',(2.74282859860853,1.2152741578159,6.5));
#8841=CARTESIAN_POINT('Origin',(2.94448637286709,1.7,6.5));
#8842=CARTESIAN_POINT('',(2.74282859860853,1.2152741578159,5.7));
#8843=CARTESIAN_POINT('',(2.74282859860853,1.2152741578159,5.7));
#8844=CARTESIAN_POINT('Origin',(2.94448637286709,1.7,5.7));
#8845=CARTESIAN_POINT('Origin',(2.94448637286709,1.7,6.5));
#8846=CARTESIAN_POINT('Origin',(0.,0.,6.5));
#8847=CARTESIAN_POINT('Origin',(2.22044604925031E-16,3.4,6.5));
#8848=CARTESIAN_POINT('',(0.318956006072958,2.98299632352941,6.5));
#8849=CARTESIAN_POINT('',(-0.318956006072958,2.98299632352941,6.5));
#8850=CARTESIAN_POINT('Origin',(0.,0.,6.5));
#8851=CARTESIAN_POINT('Origin',(2.0818995585505E-16,3.4,6.5));
#8852=CARTESIAN_POINT('Origin',(2.0818995585505E-16,3.4,5.7));
#8853=CARTESIAN_POINT('',(0.318956006072958,2.98299632352941,5.7));
#8854=CARTESIAN_POINT('',(0.318956006072958,2.98299632352941,5.7));
#8855=CARTESIAN_POINT('',(-0.318956006072958,2.98299632352941,5.7));
#8856=CARTESIAN_POINT('Origin',(2.0818995585505E-16,3.4,5.7));
#8857=CARTESIAN_POINT('',(-0.318956006072958,2.98299632352941,5.7));
#8858=CARTESIAN_POINT('Origin',(-2.94448637286709,1.7,6.5));
#8859=CARTESIAN_POINT('',(-2.42387259253558,1.76772216571351,6.5));
#8860=CARTESIAN_POINT('',(-2.74282859860853,1.2152741578159,6.5));
#8861=CARTESIAN_POINT('Origin',(0.,0.,6.5));
#8862=CARTESIAN_POINT('Origin',(-2.94448637286709,1.7,6.5));
#8863=CARTESIAN_POINT('Origin',(-2.94448637286709,1.7,5.7));
#8864=CARTESIAN_POINT('',(-2.42387259253558,1.76772216571351,5.7));
#8865=CARTESIAN_POINT('',(-2.42387259253558,1.76772216571351,5.7));
#8866=CARTESIAN_POINT('',(-2.74282859860853,1.2152741578159,5.7));
#8867=CARTESIAN_POINT('Origin',(-2.94448637286709,1.7,5.7));
#8868=CARTESIAN_POINT('',(-2.74282859860853,1.2152741578159,5.7));
#8869=CARTESIAN_POINT('Origin',(-2.94448637286709,-1.7,6.5));
#8870=CARTESIAN_POINT('',(-2.74282859860853,-1.2152741578159,6.5));
#8871=CARTESIAN_POINT('',(-2.42387259253558,-1.76772216571351,6.5));
#8872=CARTESIAN_POINT('Origin',(0.,0.,6.5));
#8873=CARTESIAN_POINT('Origin',(-2.94448637286709,-1.7,6.5));
#8874=CARTESIAN_POINT('Origin',(-2.94448637286709,-1.7,5.7));
#8875=CARTESIAN_POINT('',(-2.74282859860853,-1.2152741578159,5.7));
#8876=CARTESIAN_POINT('',(-2.74282859860853,-1.2152741578159,5.7));
#8877=CARTESIAN_POINT('',(-2.42387259253558,-1.76772216571351,5.7));
#8878=CARTESIAN_POINT('Origin',(-2.94448637286709,-1.7,5.7));
#8879=CARTESIAN_POINT('',(-2.42387259253558,-1.76772216571351,5.7));
#8880=CARTESIAN_POINT('Origin',(2.94448637286709,-1.7,5.7));
#8881=CARTESIAN_POINT('',(2.74282859860853,-1.2152741578159,6.5));
#8882=CARTESIAN_POINT('',(2.74282859860853,-1.2152741578159,5.7));
#8883=CARTESIAN_POINT('',(2.74282859860853,-1.2152741578159,5.7));
#8884=CARTESIAN_POINT('',(2.42387259253558,-1.76772216571351,6.5));
#8885=CARTESIAN_POINT('Origin',(2.94448637286709,-1.7,6.5));
#8886=CARTESIAN_POINT('',(2.42387259253558,-1.76772216571351,5.7));
#8887=CARTESIAN_POINT('',(2.42387259253558,-1.76772216571351,5.7));
#8888=CARTESIAN_POINT('Origin',(2.94448637286709,-1.7,5.7));
#8889=CARTESIAN_POINT('Origin',(2.94448637286709,-1.7,6.5));
#8890=CARTESIAN_POINT('Origin',(0.,0.,6.5));
#8891=CARTESIAN_POINT('Origin',(0.,0.,5.7));
#8892=CARTESIAN_POINT('',(-3.,-3.67394039744206E-16,9.5));
#8893=CARTESIAN_POINT('Origin',(0.,0.,9.5));
#8894=CARTESIAN_POINT('',(-3.,-3.67394039744206E-16,5.7));
#8895=CARTESIAN_POINT('',(-3.,-3.67394039744206E-16,5.7));
#8896=CARTESIAN_POINT('Origin',(0.,0.,5.7));
#8897=CARTESIAN_POINT('Origin',(0.,0.,5.7));
#8898=CARTESIAN_POINT('Origin',(0.,0.,5.7));
#8899=CARTESIAN_POINT('Origin',(0.,0.,5.7));
#8900=CARTESIAN_POINT('Origin',(0.,0.,5.7));
#8901=CARTESIAN_POINT('Origin',(0.,0.,5.7));
#8902=CARTESIAN_POINT('Origin',(0.,0.,5.7));
#8903=CARTESIAN_POINT('Origin',(-6.2456986756515E-16,-3.4,4.9));
#8904=CARTESIAN_POINT('',(-0.275000000000001,-3.4,5.1));
#8905=CARTESIAN_POINT('Origin',(-6.2456986756515E-16,-3.4,5.1));
#8906=CARTESIAN_POINT('',(-0.275000000000001,-3.4,5.7));
#8907=CARTESIAN_POINT('',(-0.275000000000001,-3.4,4.9));
#8908=CARTESIAN_POINT('Origin',(-6.2456986756515E-16,-3.4,5.7));
#8909=CARTESIAN_POINT('Origin',(2.94448637286709,1.7,4.9));
#8910=CARTESIAN_POINT('',(2.66948637286709,1.7,5.1));
#8911=CARTESIAN_POINT('Origin',(2.94448637286709,1.7,5.1));
#8912=CARTESIAN_POINT('',(2.66948637286709,1.7,5.7));
#8913=CARTESIAN_POINT('',(2.66948637286709,1.7,4.9));
#8914=CARTESIAN_POINT('Origin',(2.94448637286709,1.7,5.7));
#8915=CARTESIAN_POINT('Origin',(2.0818995585505E-16,3.4,4.9));
#8916=CARTESIAN_POINT('',(-0.275,3.4,5.1));
#8917=CARTESIAN_POINT('Origin',(2.0818995585505E-16,3.4,5.1));
#8918=CARTESIAN_POINT('',(-0.275,3.4,5.7));
#8919=CARTESIAN_POINT('',(-0.275,3.4,4.9));
#8920=CARTESIAN_POINT('Origin',(2.0818995585505E-16,3.4,5.7));
#8921=CARTESIAN_POINT('Origin',(-2.94448637286709,1.7,4.9));
#8922=CARTESIAN_POINT('',(-3.21948637286709,1.7,5.1));
#8923=CARTESIAN_POINT('Origin',(-2.94448637286709,1.7,5.1));
#8924=CARTESIAN_POINT('',(-3.21948637286709,1.7,5.7));
#8925=CARTESIAN_POINT('',(-3.21948637286709,1.7,4.9));
#8926=CARTESIAN_POINT('Origin',(-2.94448637286709,1.7,5.7));
#8927=CARTESIAN_POINT('Origin',(-2.94448637286709,-1.7,4.9));
#8928=CARTESIAN_POINT('',(-3.21948637286709,-1.7,5.1));
#8929=CARTESIAN_POINT('Origin',(-2.94448637286709,-1.7,5.1));
#8930=CARTESIAN_POINT('',(-3.21948637286709,-1.7,5.7));
#8931=CARTESIAN_POINT('',(-3.21948637286709,-1.7,4.9));
#8932=CARTESIAN_POINT('Origin',(-2.94448637286709,-1.7,5.7));
#8933=CARTESIAN_POINT('Origin',(2.94448637286709,-1.7,4.9));
#8934=CARTESIAN_POINT('',(2.66948637286709,-1.7,5.1));
#8935=CARTESIAN_POINT('Origin',(2.94448637286709,-1.7,5.1));
#8936=CARTESIAN_POINT('',(2.66948637286709,-1.7,5.7));
#8937=CARTESIAN_POINT('',(2.66948637286709,-1.7,4.9));
#8938=CARTESIAN_POINT('Origin',(2.94448637286709,-1.7,5.7));
#8939=CARTESIAN_POINT('Origin',(0.,0.,8.7));
#8940=CARTESIAN_POINT('',(-0.34,-4.163799117101E-17,8.8));
#8941=CARTESIAN_POINT('Origin',(0.,0.,8.8));
#8942=CARTESIAN_POINT('',(-0.34,4.163799117101E-17,9.5));
#8943=CARTESIAN_POINT('',(-0.34,-4.163799117101E-17,8.7));
#8944=CARTESIAN_POINT('Origin',(0.,0.,9.5));
#8945=CARTESIAN_POINT('Origin',(0.,0.,5.));
#8946=CARTESIAN_POINT('',(-2.5,-3.06161699786838E-16,5.1));
#8947=CARTESIAN_POINT('Origin',(0.,0.,5.1));
#8948=CARTESIAN_POINT('',(-2.5,-3.06161699786838E-16,8.8));
#8949=CARTESIAN_POINT('',(-2.5,-3.06161699786838E-16,5.));
#8950=CARTESIAN_POINT('Origin',(0.,0.,8.8));
#8951=CARTESIAN_POINT('Origin',(0.,0.,8.8));
#8952=CARTESIAN_POINT('Origin',(0.,0.,9.5));
#8953=CARTESIAN_POINT('Origin',(0.,0.,5.1));
#8954=CARTESIAN_POINT('',(-4.,-4.89858719658941E-16,5.7));
#8955=CARTESIAN_POINT('Origin',(0.,0.,5.7));
#8956=CARTESIAN_POINT('',(-4.,-4.89858719658941E-16,5.1));
#8957=CARTESIAN_POINT('',(-4.,-4.89858719658941E-16,5.1));
#8958=CARTESIAN_POINT('Origin',(0.,0.,5.1));
#8959=CARTESIAN_POINT('Origin',(0.,0.,5.7));
#8960=CARTESIAN_POINT('Origin',(0.,0.,5.1));
#10229=UNCERTAINTY_MEASURE_WITH_UNIT(LENGTH_MEASURE(0.001),#10267,
'DISTANCE_ACCURACY_VALUE',
'Maximum model space distance between geometric entities at asserted c
onnectivities');
#10241=UNCERTAINTY_MEASURE_WITH_UNIT(LENGTH_MEASURE(0.001),#10267,
'DISTANCE_ACCURACY_VALUE',
'Maximum model space distance between geometric entities at asserted c
onnectivities');
#10254=(
GEOMETRIC_REPRESENTATION_CONTEXT(3)
GLOBAL_UNCERTAINTY_ASSIGNED_CONTEXT((#10229))
GLOBAL_UNIT_ASSIGNED_CONTEXT((#10267,#10269,#10270))
REPRESENTATION_CONTEXT('','3D')
);
#10266=(
GEOMETRIC_REPRESENTATION_CONTEXT(3)
GLOBAL_UNCERTAINTY_ASSIGNED_CONTEXT((#10241))
GLOBAL_UNIT_ASSIGNED_CONTEXT((#10267,#10269,#10270))
REPRESENTATION_CONTEXT('','3D')
);
#10267=(
LENGTH_UNIT()
NAMED_UNIT(*)
SI_UNIT(.CENTI.,.METRE.)
);
#10269=(
NAMED_UNIT(*)
PLANE_ANGLE_UNIT()
SI_UNIT($,.RADIAN.)
);
#10270=(
NAMED_UNIT(*)
SI_UNIT($,.STERADIAN.)
SOLID_ANGLE_UNIT()
);
#10283=SHAPE_DEFINITION_REPRESENTATION(#10307,#10366);
#10307=PRODUCT_DEFINITION_SHAPE('',$,#10391);
#10366=SHAPE_REPRESENTATION('',(#5306),#10254);
#10378=PRODUCT_DEFINITION_CONTEXT('part definition',#10452,'design');
#10391=PRODUCT_DEFINITION('Bonnet','Bonnet',#10415,#10378);
#10415=PRODUCT_DEFINITION_FORMATION('',$,#10466);
#10452=APPLICATION_CONTEXT(
'Core Data for Automotive Mechanical Design Process');
#10453=PRODUCT_CONTEXT('part definition',#10452,'mechanical');
#10466=PRODUCT('Bonnet','Bonnet','Bonnet',(#10453));
#10534=COLOUR_RGB('Sky Blue',0.24,0.69,0.87);
#10535=FILL_AREA_STYLE_COLOUR('',#10534);
#10536=FILL_AREA_STYLE('',(#10535));
#10537=SURFACE_STYLE_FILL_AREA(#10536);
#10538=SURFACE_SIDE_STYLE('',(#10537));
#10539=SURFACE_STYLE_USAGE(.BOTH.,#10538);
#10540=PRESENTATION_STYLE_ASSIGNMENT((#10539));
ENDSEC;
END-ISO-10303-21;
